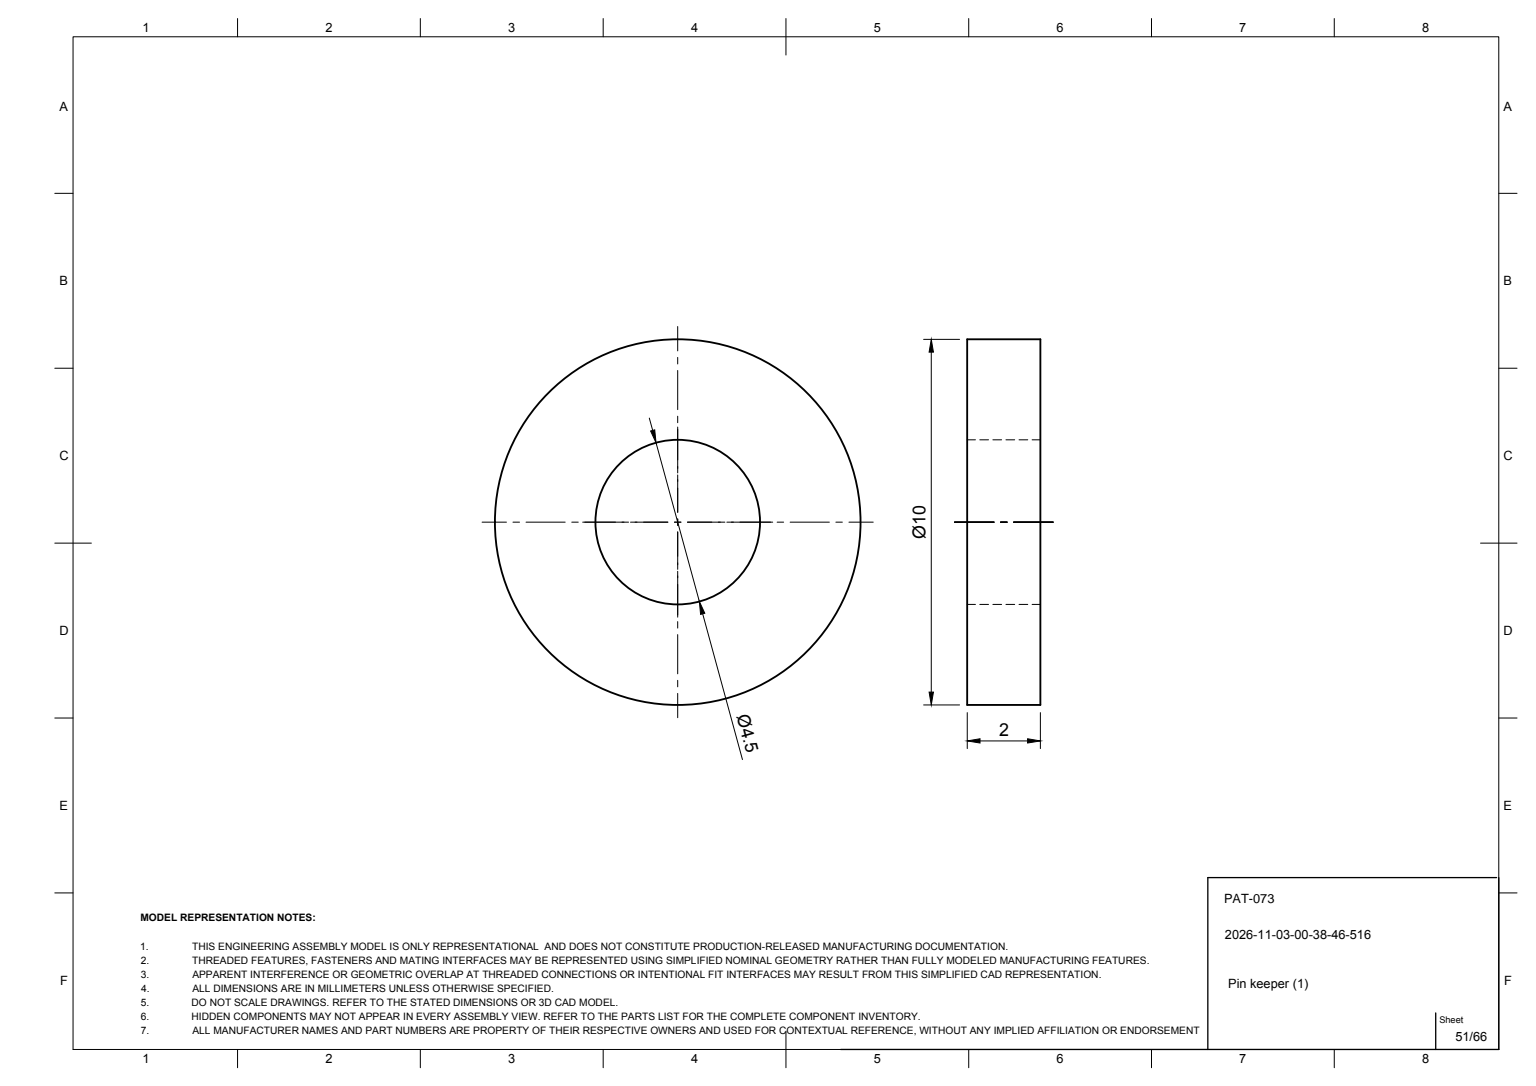
ISO-10303-21;
HEADER;
/* Generated by software containing ST-Developer
 * from STEP Tools, Inc. (www.steptools.com) 
 */

FILE_DESCRIPTION(
/* description */ ('Manual piston pump'),
/* implementation_level */ '2;1');

FILE_NAME(
/* name */ 'Pin keeper (1).step',
/* time_stamp */ '2026-11-02T16:54:23-08:00',
/* author */ (''),
/* organization */ (''),
/* preprocessor_version */ 'ST-DEVELOPER v20.2',
/* originating_system */ 'Autodesk Translation Framework v15.17.0.0',
/* authorisation */ '');

FILE_SCHEMA (('AUTOMOTIVE_DESIGN { 1 0 10303 214 3 1 1 }'));
ENDSEC;

DATA;
#10=MECHANICAL_DESIGN_GEOMETRIC_PRESENTATION_REPRESENTATION('',(#742),#19043);
#608=SHAPE_REPRESENTATION_RELATIONSHIP('SRR','None',#19357,#671);
#671=ADVANCED_BREP_SHAPE_REPRESENTATION('',(#811),#19024);
#742=STYLED_ITEM('',(#19661),#811);
#811=MANIFOLD_SOLID_BREP('Body1',#9529);
#1017=FACE_BOUND('',#2510,.T.);
#1018=FACE_BOUND('',#2512,.T.);
#1252=CYLINDRICAL_SURFACE('',#11152,0.225);
#1253=CYLINDRICAL_SURFACE('',#11155,0.5);
#1742=FACE_OUTER_BOUND('',#2507,.T.);
#1743=FACE_OUTER_BOUND('',#2508,.T.);
#1744=FACE_OUTER_BOUND('',#2509,.T.);
#1745=FACE_OUTER_BOUND('',#2511,.T.);
#2507=EDGE_LOOP('',(#8091,#8092,#8093,#8094));
#2508=EDGE_LOOP('',(#8095,#8096,#8097,#8098));
#2509=EDGE_LOOP('',(#8099));
#2510=EDGE_LOOP('',(#8100));
#2511=EDGE_LOOP('',(#8101));
#2512=EDGE_LOOP('',(#8102));
#3058=CIRCLE('',#11153,0.225);
#3059=CIRCLE('',#11154,0.225);
#3060=CIRCLE('',#11156,0.5);
#3061=CIRCLE('',#11157,0.5);
#3613=LINE('',#18144,#4217);
#3614=LINE('',#18150,#4218);
#4217=VECTOR('',#13783,0.225);
#4218=VECTOR('',#13790,0.5);
#4966=VERTEX_POINT('',#18141);
#4967=VERTEX_POINT('',#18143);
#4968=VERTEX_POINT('',#18147);
#4969=VERTEX_POINT('',#18149);
#6032=EDGE_CURVE('',#4966,#4966,#3058,.T.);
#6033=EDGE_CURVE('',#4966,#4967,#3613,.T.);
#6034=EDGE_CURVE('',#4967,#4967,#3059,.T.);
#6035=EDGE_CURVE('',#4968,#4968,#3060,.T.);
#6036=EDGE_CURVE('',#4968,#4969,#3614,.T.);
#6037=EDGE_CURVE('',#4969,#4969,#3061,.T.);
#8091=ORIENTED_EDGE('',*,*,#6032,.F.);
#8092=ORIENTED_EDGE('',*,*,#6033,.T.);
#8093=ORIENTED_EDGE('',*,*,#6034,.T.);
#8094=ORIENTED_EDGE('',*,*,#6033,.F.);
#8095=ORIENTED_EDGE('',*,*,#6035,.F.);
#8096=ORIENTED_EDGE('',*,*,#6036,.T.);
#8097=ORIENTED_EDGE('',*,*,#6037,.T.);
#8098=ORIENTED_EDGE('',*,*,#6036,.F.);
#8099=ORIENTED_EDGE('',*,*,#6035,.T.);
#8100=ORIENTED_EDGE('',*,*,#6032,.T.);
#8101=ORIENTED_EDGE('',*,*,#6037,.F.);
#8102=ORIENTED_EDGE('',*,*,#6034,.F.);
#8821=PLANE('',#11158);
#8822=PLANE('',#11159);
#9347=ADVANCED_FACE('',(#1742),#1252,.F.);
#9348=ADVANCED_FACE('',(#1743),#1253,.T.);
#9349=ADVANCED_FACE('',(#1744,#1017),#8821,.T.);
#9350=ADVANCED_FACE('',(#1745,#1018),#8822,.F.);
#9529=CLOSED_SHELL('',(#9347,#9348,#9349,#9350));
#11151=AXIS2_PLACEMENT_3D('',#18139,#13777,#13778);
#11152=AXIS2_PLACEMENT_3D('',#18140,#13779,#13780);
#11153=AXIS2_PLACEMENT_3D('',#18142,#13781,#13782);
#11154=AXIS2_PLACEMENT_3D('',#18145,#13784,#13785);
#11155=AXIS2_PLACEMENT_3D('',#18146,#13786,#13787);
#11156=AXIS2_PLACEMENT_3D('',#18148,#13788,#13789);
#11157=AXIS2_PLACEMENT_3D('',#18151,#13791,#13792);
#11158=AXIS2_PLACEMENT_3D('',#18152,#13793,#13794);
#11159=AXIS2_PLACEMENT_3D('',#18153,#13795,#13796);
#13777=DIRECTION('axis',(0.,0.,1.));
#13778=DIRECTION('refdir',(1.,0.,0.));
#13779=DIRECTION('center_axis',(1.,0.,0.));
#13780=DIRECTION('ref_axis',(0.,0.,-1.));
#13781=DIRECTION('center_axis',(-1.,0.,0.));
#13782=DIRECTION('ref_axis',(0.,0.,-1.));
#13783=DIRECTION('',(-1.,0.,0.));
#13784=DIRECTION('center_axis',(-1.,0.,0.));
#13785=DIRECTION('ref_axis',(0.,0.,-1.));
#13786=DIRECTION('center_axis',(1.,0.,0.));
#13787=DIRECTION('ref_axis',(0.,0.,-1.));
#13788=DIRECTION('center_axis',(1.,0.,0.));
#13789=DIRECTION('ref_axis',(0.,0.,-1.));
#13790=DIRECTION('',(-1.,0.,0.));
#13791=DIRECTION('center_axis',(1.,0.,0.));
#13792=DIRECTION('ref_axis',(0.,0.,-1.));
#13793=DIRECTION('center_axis',(1.,0.,0.));
#13794=DIRECTION('ref_axis',(0.,0.,-1.));
#13795=DIRECTION('center_axis',(1.,0.,0.));
#13796=DIRECTION('ref_axis',(0.,0.,-1.));
#18139=CARTESIAN_POINT('',(0.,0.,0.));
#18140=CARTESIAN_POINT('Origin',(1.2,-6.1,4.5));
#18141=CARTESIAN_POINT('',(1.4,-6.1,4.725));
#18142=CARTESIAN_POINT('Origin',(1.4,-6.1,4.5));
#18143=CARTESIAN_POINT('',(1.2,-6.1,4.725));
#18144=CARTESIAN_POINT('',(1.2,-6.1,4.725));
#18145=CARTESIAN_POINT('Origin',(1.2,-6.1,4.5));
#18146=CARTESIAN_POINT('Origin',(1.2,-6.1,4.5));
#18147=CARTESIAN_POINT('',(1.4,-6.1,5.));
#18148=CARTESIAN_POINT('Origin',(1.4,-6.1,4.5));
#18149=CARTESIAN_POINT('',(1.2,-6.1,5.));
#18150=CARTESIAN_POINT('',(1.2,-6.1,5.));
#18151=CARTESIAN_POINT('Origin',(1.2,-6.1,4.5));
#18152=CARTESIAN_POINT('Origin',(1.4,-6.1,4.5));
#18153=CARTESIAN_POINT('Origin',(1.2,-6.1,4.5));
#18953=UNCERTAINTY_MEASURE_WITH_UNIT(LENGTH_MEASURE(0.001),#19044,
'DISTANCE_ACCURACY_VALUE',
'Maximum model space distance between geometric entities at asserted c
onnectivities');
#18972=UNCERTAINTY_MEASURE_WITH_UNIT(LENGTH_MEASURE(0.001),#19044,
'DISTANCE_ACCURACY_VALUE',
'Maximum model space distance between geometric entities at asserted c
onnectivities');
#19024=(
GEOMETRIC_REPRESENTATION_CONTEXT(3)
GLOBAL_UNCERTAINTY_ASSIGNED_CONTEXT((#18953))
GLOBAL_UNIT_ASSIGNED_CONTEXT((#19044,#19046,#19047))
REPRESENTATION_CONTEXT('','3D')
);
#19043=(
GEOMETRIC_REPRESENTATION_CONTEXT(3)
GLOBAL_UNCERTAINTY_ASSIGNED_CONTEXT((#18972))
GLOBAL_UNIT_ASSIGNED_CONTEXT((#19044,#19046,#19047))
REPRESENTATION_CONTEXT('','3D')
);
#19044=(
LENGTH_UNIT()
NAMED_UNIT(*)
SI_UNIT(.CENTI.,.METRE.)
);
#19046=(
NAMED_UNIT(*)
PLANE_ANGLE_UNIT()
SI_UNIT($,.RADIAN.)
);
#19047=(
NAMED_UNIT(*)
SI_UNIT($,.STERADIAN.)
SOLID_ANGLE_UNIT()
);
#19099=SHAPE_DEFINITION_REPRESENTATION(#19176,#19357);
#19176=PRODUCT_DEFINITION_SHAPE('',$,#19428);
#19357=SHAPE_REPRESENTATION('',(#11151),#19024);
#19376=PRODUCT_DEFINITION_CONTEXT('part definition',#19588,'design');
#19428=PRODUCT_DEFINITION('2026-11-03-00-38-46-516','Pin keeper (1)',#19498,
#19376);
#19498=PRODUCT_DEFINITION_FORMATION('',$,#19641);
#19588=APPLICATION_CONTEXT(
'Core Data for Automotive Mechanical Design Process');
#19589=PRODUCT_CONTEXT('part definition',#19588,'mechanical');
#19641=PRODUCT('2026-11-03-00-38-46-516','Pin keeper (1)','Pin keeper',
(#19589));
#19661=PRESENTATION_STYLE_ASSIGNMENT((#19667));
#19667=SURFACE_STYLE_USAGE(.BOTH.,#19673);
#19673=SURFACE_SIDE_STYLE('',(#19679));
#19679=SURFACE_STYLE_FILL_AREA(#19685);
#19685=FILL_AREA_STYLE('CAD Library Painted - Engineering blue',(#19691));
#19691=FILL_AREA_STYLE_COLOUR('CAD Library Painted - Engineering blue',
#19697);
#19697=COLOUR_RGB('CAD Library Painted - Engineering blue',0.12156862745098,
0.356862745098039,0.6);
ENDSEC;
END-ISO-10303-21;
